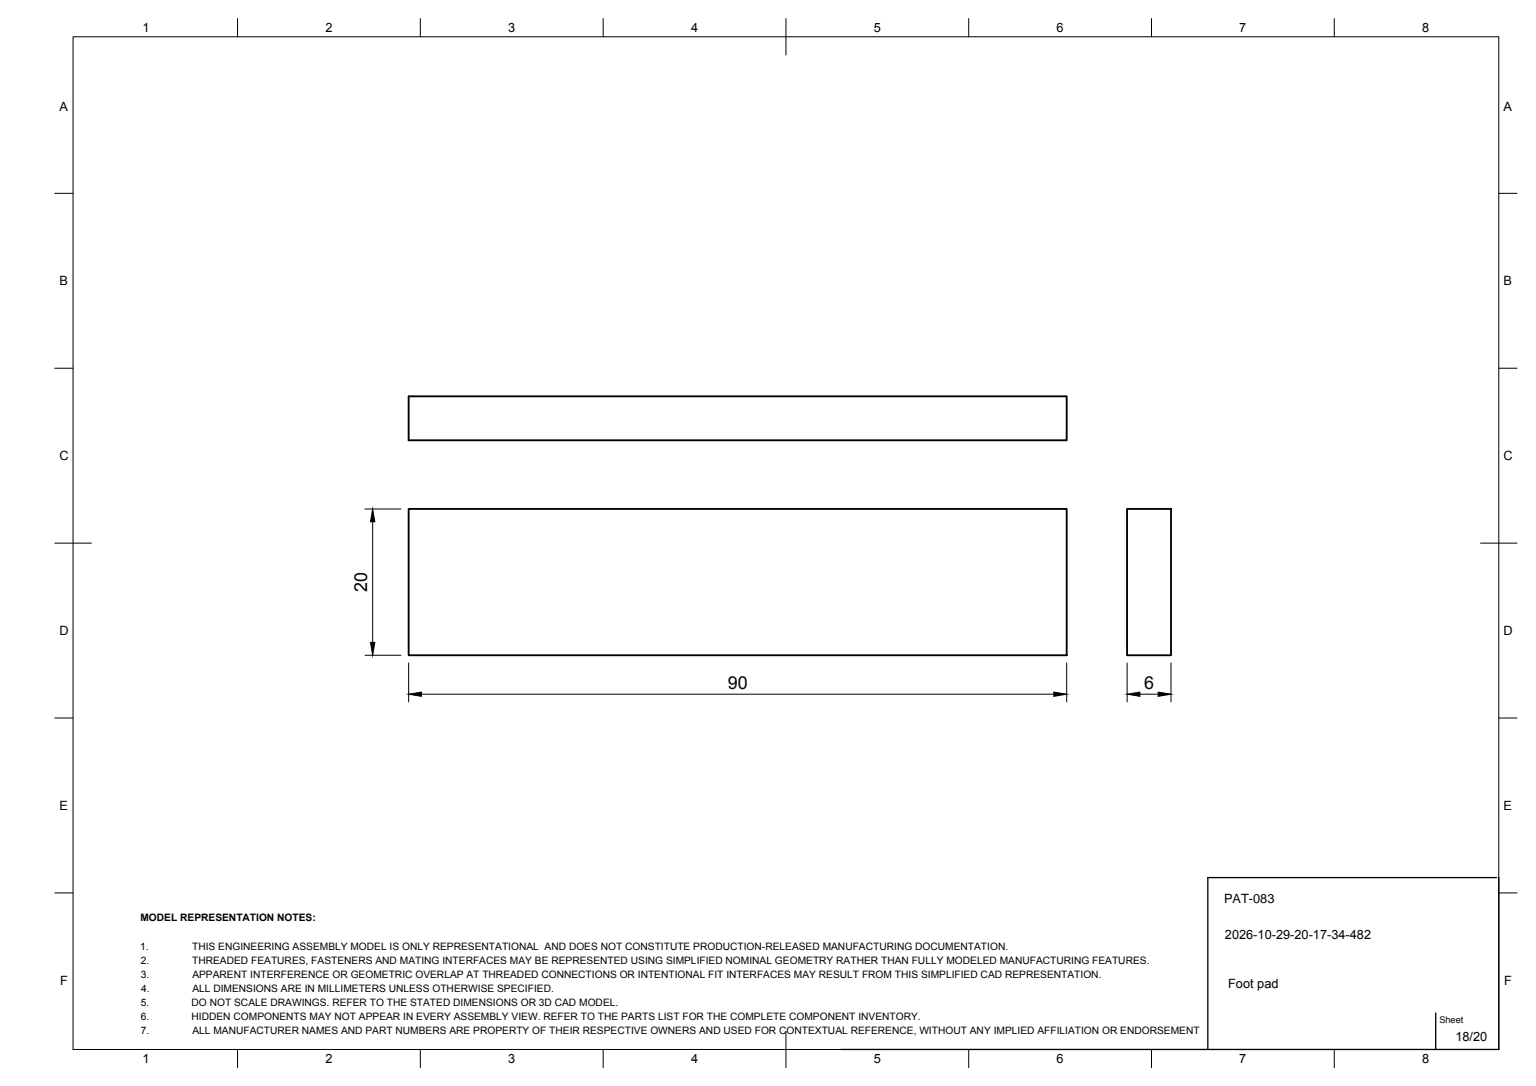
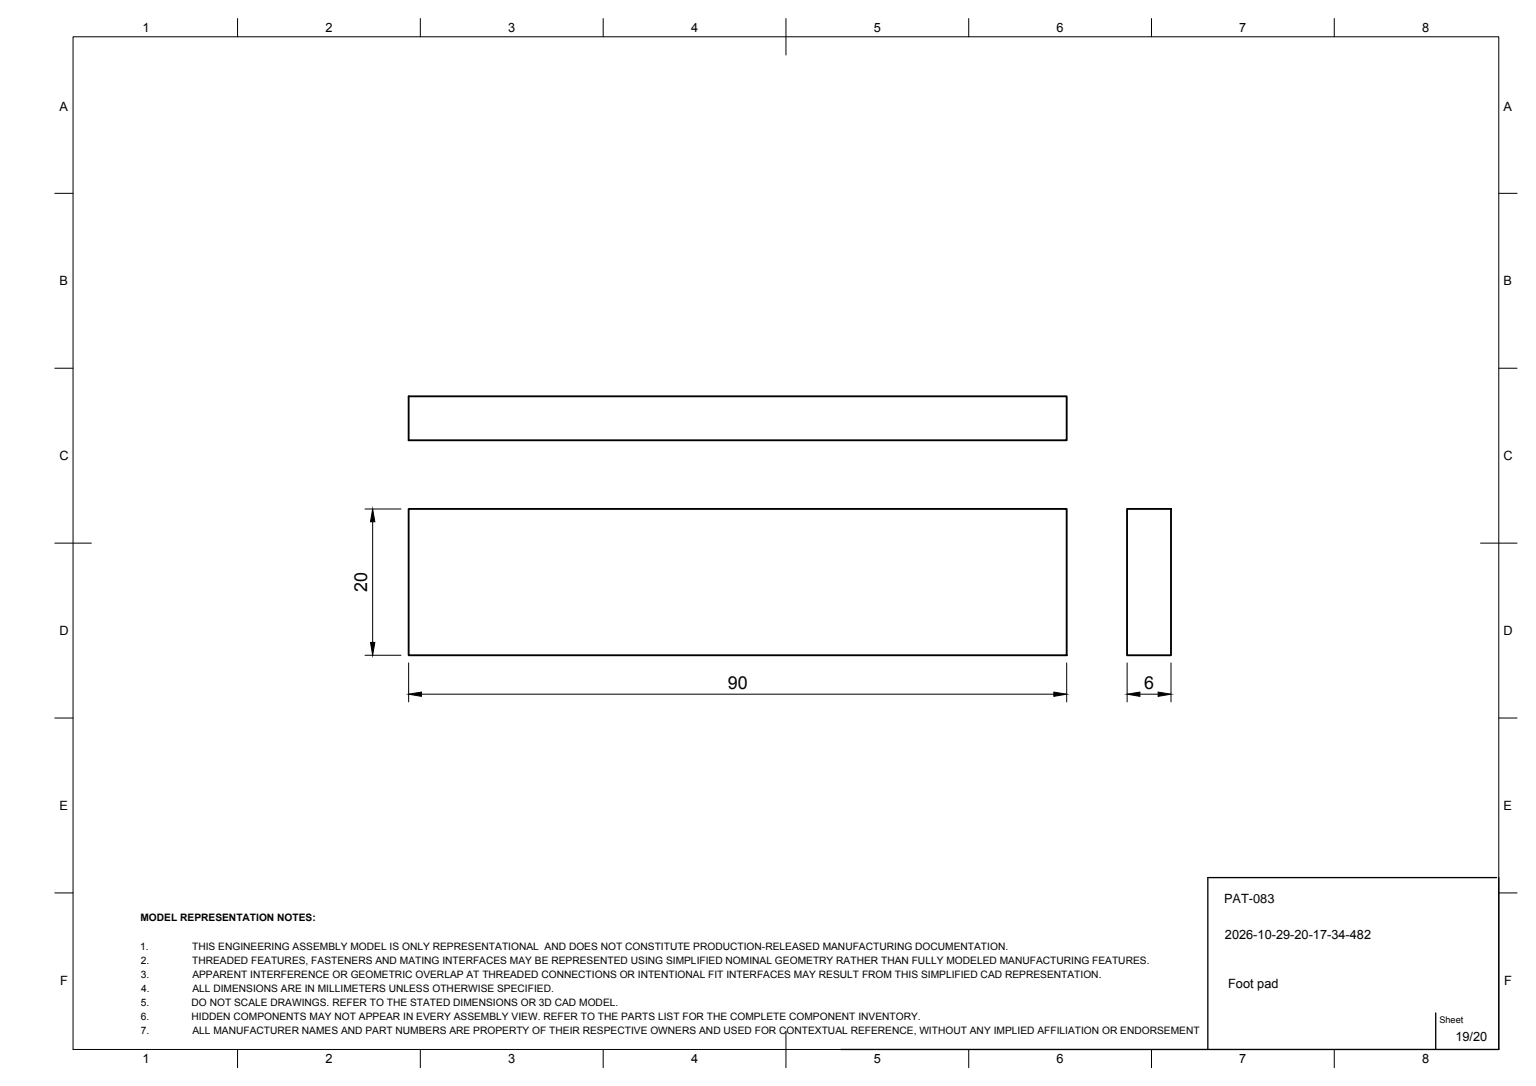
ISO-10303-21;
HEADER;
/* Generated by software containing ST-Developer
 * from STEP Tools, Inc. (www.steptools.com) 
 */

FILE_DESCRIPTION(
/* description */ ('PAT-083'),
/* implementation_level */ '2;1');

FILE_NAME(
/* name */ 'Foot pad.step',
/* time_stamp */ '2026-10-29T20:18:00-07:00',
/* author */ (''),
/* organization */ (''),
/* preprocessor_version */ 'ST-DEVELOPER v20.2',
/* originating_system */ 'Autodesk Translation Framework v15.17.0.0',
/* authorisation */ '');

FILE_SCHEMA (('AUTOMOTIVE_DESIGN { 1 0 10303 214 3 1 1 }'));
ENDSEC;

DATA;
#10=MECHANICAL_DESIGN_GEOMETRIC_PRESENTATION_REPRESENTATION('',(#245),#8428);
#197=SHAPE_REPRESENTATION_RELATIONSHIP('SRR','None',#8531,#221);
#221=ADVANCED_BREP_SHAPE_REPRESENTATION('',(#269),#8420);
#245=STYLED_ITEM('',(#8698),#269);
#269=MANIFOLD_SOLID_BREP('Body1',#3691);
#432=PLANE('',#4274);
#433=PLANE('',#4275);
#434=PLANE('',#4276);
#435=PLANE('',#4277);
#436=PLANE('',#4278);
#437=PLANE('',#4279);
#640=FACE_OUTER_BOUND('',#943,.T.);
#641=FACE_OUTER_BOUND('',#944,.T.);
#642=FACE_OUTER_BOUND('',#945,.T.);
#643=FACE_OUTER_BOUND('',#946,.T.);
#644=FACE_OUTER_BOUND('',#947,.T.);
#645=FACE_OUTER_BOUND('',#948,.T.);
#943=EDGE_LOOP('',(#3014,#3015,#3016,#3017));
#944=EDGE_LOOP('',(#3018,#3019,#3020,#3021));
#945=EDGE_LOOP('',(#3022,#3023,#3024,#3025));
#946=EDGE_LOOP('',(#3026,#3027,#3028,#3029));
#947=EDGE_LOOP('',(#3030,#3031,#3032,#3033));
#948=EDGE_LOOP('',(#3034,#3035,#3036,#3037));
#1159=LINE('',#7943,#1403);
#1160=LINE('',#7945,#1404);
#1161=LINE('',#7947,#1405);
#1162=LINE('',#7948,#1406);
#1163=LINE('',#7951,#1407);
#1164=LINE('',#7953,#1408);
#1165=LINE('',#7954,#1409);
#1166=LINE('',#7957,#1410);
#1167=LINE('',#7959,#1411);
#1168=LINE('',#7960,#1412);
#1169=LINE('',#7962,#1413);
#1170=LINE('',#7963,#1414);
#1403=VECTOR('',#5171,1.);
#1404=VECTOR('',#5172,1.);
#1405=VECTOR('',#5173,1.);
#1406=VECTOR('',#5174,1.);
#1407=VECTOR('',#5177,1.);
#1408=VECTOR('',#5178,1.);
#1409=VECTOR('',#5179,1.);
#1410=VECTOR('',#5182,1.);
#1411=VECTOR('',#5183,1.);
#1412=VECTOR('',#5184,1.);
#1413=VECTOR('',#5187,1.);
#1414=VECTOR('',#5188,1.);
#1893=VERTEX_POINT('',#7941);
#1894=VERTEX_POINT('',#7942);
#1895=VERTEX_POINT('',#7944);
#1896=VERTEX_POINT('',#7946);
#1897=VERTEX_POINT('',#7950);
#1898=VERTEX_POINT('',#7952);
#1899=VERTEX_POINT('',#7956);
#1900=VERTEX_POINT('',#7958);
#2283=EDGE_CURVE('',#1893,#1894,#1159,.T.);
#2284=EDGE_CURVE('',#1894,#1895,#1160,.T.);
#2285=EDGE_CURVE('',#1896,#1895,#1161,.T.);
#2286=EDGE_CURVE('',#1893,#1896,#1162,.T.);
#2287=EDGE_CURVE('',#1897,#1893,#1163,.T.);
#2288=EDGE_CURVE('',#1898,#1896,#1164,.T.);
#2289=EDGE_CURVE('',#1897,#1898,#1165,.T.);
#2290=EDGE_CURVE('',#1899,#1897,#1166,.T.);
#2291=EDGE_CURVE('',#1900,#1898,#1167,.T.);
#2292=EDGE_CURVE('',#1899,#1900,#1168,.T.);
#2293=EDGE_CURVE('',#1894,#1899,#1169,.T.);
#2294=EDGE_CURVE('',#1895,#1900,#1170,.T.);
#3014=ORIENTED_EDGE('',*,*,#2283,.T.);
#3015=ORIENTED_EDGE('',*,*,#2284,.T.);
#3016=ORIENTED_EDGE('',*,*,#2285,.F.);
#3017=ORIENTED_EDGE('',*,*,#2286,.F.);
#3018=ORIENTED_EDGE('',*,*,#2287,.T.);
#3019=ORIENTED_EDGE('',*,*,#2286,.T.);
#3020=ORIENTED_EDGE('',*,*,#2288,.F.);
#3021=ORIENTED_EDGE('',*,*,#2289,.F.);
#3022=ORIENTED_EDGE('',*,*,#2290,.T.);
#3023=ORIENTED_EDGE('',*,*,#2289,.T.);
#3024=ORIENTED_EDGE('',*,*,#2291,.F.);
#3025=ORIENTED_EDGE('',*,*,#2292,.F.);
#3026=ORIENTED_EDGE('',*,*,#2293,.T.);
#3027=ORIENTED_EDGE('',*,*,#2292,.T.);
#3028=ORIENTED_EDGE('',*,*,#2294,.F.);
#3029=ORIENTED_EDGE('',*,*,#2284,.F.);
#3030=ORIENTED_EDGE('',*,*,#2294,.T.);
#3031=ORIENTED_EDGE('',*,*,#2291,.T.);
#3032=ORIENTED_EDGE('',*,*,#2288,.T.);
#3033=ORIENTED_EDGE('',*,*,#2285,.T.);
#3034=ORIENTED_EDGE('',*,*,#2293,.F.);
#3035=ORIENTED_EDGE('',*,*,#2283,.F.);
#3036=ORIENTED_EDGE('',*,*,#2287,.F.);
#3037=ORIENTED_EDGE('',*,*,#2290,.F.);
#3587=ADVANCED_FACE('',(#640),#432,.T.);
#3588=ADVANCED_FACE('',(#641),#433,.T.);
#3589=ADVANCED_FACE('',(#642),#434,.T.);
#3590=ADVANCED_FACE('',(#643),#435,.T.);
#3591=ADVANCED_FACE('',(#644),#436,.T.);
#3592=ADVANCED_FACE('',(#645),#437,.F.);
#3691=CLOSED_SHELL('',(#3587,#3588,#3589,#3590,#3591,#3592));
#4273=AXIS2_PLACEMENT_3D('',#7939,#5167,#5168);
#4274=AXIS2_PLACEMENT_3D('',#7940,#5169,#5170);
#4275=AXIS2_PLACEMENT_3D('',#7949,#5175,#5176);
#4276=AXIS2_PLACEMENT_3D('',#7955,#5180,#5181);
#4277=AXIS2_PLACEMENT_3D('',#7961,#5185,#5186);
#4278=AXIS2_PLACEMENT_3D('',#7964,#5189,#5190);
#4279=AXIS2_PLACEMENT_3D('',#7965,#5191,#5192);
#5167=DIRECTION('axis',(0.,0.,1.));
#5168=DIRECTION('refdir',(1.,0.,0.));
#5169=DIRECTION('center_axis',(0.,1.,0.));
#5170=DIRECTION('ref_axis',(-1.,0.,0.));
#5171=DIRECTION('',(-1.,0.,0.));
#5172=DIRECTION('',(0.,0.,1.));
#5173=DIRECTION('',(-1.,0.,0.));
#5174=DIRECTION('',(0.,0.,1.));
#5175=DIRECTION('center_axis',(1.,0.,0.));
#5176=DIRECTION('ref_axis',(0.,1.,0.));
#5177=DIRECTION('',(0.,1.,0.));
#5178=DIRECTION('',(0.,1.,0.));
#5179=DIRECTION('',(0.,0.,1.));
#5180=DIRECTION('center_axis',(0.,-1.,0.));
#5181=DIRECTION('ref_axis',(1.,0.,0.));
#5182=DIRECTION('',(1.,0.,0.));
#5183=DIRECTION('',(1.,0.,0.));
#5184=DIRECTION('',(0.,0.,1.));
#5185=DIRECTION('center_axis',(-1.,0.,0.));
#5186=DIRECTION('ref_axis',(0.,-1.,0.));
#5187=DIRECTION('',(0.,-1.,0.));
#5188=DIRECTION('',(0.,-1.,0.));
#5189=DIRECTION('center_axis',(0.,0.,1.));
#5190=DIRECTION('ref_axis',(1.,0.,0.));
#5191=DIRECTION('center_axis',(0.,0.,1.));
#5192=DIRECTION('ref_axis',(1.,0.,0.));
#7939=CARTESIAN_POINT('',(0.,0.,0.));
#7940=CARTESIAN_POINT('Origin',(-4.,4.5,-0.6));
#7941=CARTESIAN_POINT('',(-4.,4.5,-0.6));
#7942=CARTESIAN_POINT('',(-6.,4.5,-0.6));
#7943=CARTESIAN_POINT('',(-4.,4.5,-0.6));
#7944=CARTESIAN_POINT('',(-6.,4.5,0.));
#7945=CARTESIAN_POINT('',(-6.,4.5,-0.6));
#7946=CARTESIAN_POINT('',(-4.,4.5,0.));
#7947=CARTESIAN_POINT('',(-4.,4.5,0.));
#7948=CARTESIAN_POINT('',(-4.,4.5,-0.6));
#7949=CARTESIAN_POINT('Origin',(-4.,-4.5,-0.6));
#7950=CARTESIAN_POINT('',(-4.,-4.5,-0.6));
#7951=CARTESIAN_POINT('',(-4.,-4.5,-0.6));
#7952=CARTESIAN_POINT('',(-4.,-4.5,0.));
#7953=CARTESIAN_POINT('',(-4.,-4.5,0.));
#7954=CARTESIAN_POINT('',(-4.,-4.5,-0.6));
#7955=CARTESIAN_POINT('Origin',(-6.,-4.5,-0.6));
#7956=CARTESIAN_POINT('',(-6.,-4.5,-0.6));
#7957=CARTESIAN_POINT('',(-6.,-4.5,-0.6));
#7958=CARTESIAN_POINT('',(-6.,-4.5,0.));
#7959=CARTESIAN_POINT('',(-6.,-4.5,0.));
#7960=CARTESIAN_POINT('',(-6.,-4.5,-0.6));
#7961=CARTESIAN_POINT('Origin',(-6.,4.5,-0.6));
#7962=CARTESIAN_POINT('',(-6.,4.5,-0.6));
#7963=CARTESIAN_POINT('',(-6.,4.5,0.));
#7964=CARTESIAN_POINT('Origin',(-5.,0.,0.));
#7965=CARTESIAN_POINT('Origin',(-5.,0.,-0.6));
#8394=UNCERTAINTY_MEASURE_WITH_UNIT(LENGTH_MEASURE(0.001),#8429,
'DISTANCE_ACCURACY_VALUE',
'Maximum model space distance between geometric entities at asserted c
onnectivities');
#8402=UNCERTAINTY_MEASURE_WITH_UNIT(LENGTH_MEASURE(0.001),#8429,
'DISTANCE_ACCURACY_VALUE',
'Maximum model space distance between geometric entities at asserted c
onnectivities');
#8420=(
GEOMETRIC_REPRESENTATION_CONTEXT(3)
GLOBAL_UNCERTAINTY_ASSIGNED_CONTEXT((#8394))
GLOBAL_UNIT_ASSIGNED_CONTEXT((#8429,#8431,#8432))
REPRESENTATION_CONTEXT('','3D')
);
#8428=(
GEOMETRIC_REPRESENTATION_CONTEXT(3)
GLOBAL_UNCERTAINTY_ASSIGNED_CONTEXT((#8402))
GLOBAL_UNIT_ASSIGNED_CONTEXT((#8429,#8431,#8432))
REPRESENTATION_CONTEXT('','3D')
);
#8429=(
LENGTH_UNIT()
NAMED_UNIT(*)
SI_UNIT(.CENTI.,.METRE.)
);
#8431=(
NAMED_UNIT(*)
PLANE_ANGLE_UNIT()
SI_UNIT($,.RADIAN.)
);
#8432=(
NAMED_UNIT(*)
SI_UNIT($,.STERADIAN.)
SOLID_ANGLE_UNIT()
);
#8450=SHAPE_DEFINITION_REPRESENTATION(#8475,#8531);
#8475=PRODUCT_DEFINITION_SHAPE('',$,#8557);
#8531=SHAPE_REPRESENTATION('',(#4273),#8420);
#8539=PRODUCT_DEFINITION_CONTEXT('part definition',#8616,'design');
#8557=PRODUCT_DEFINITION('Foot pad','Foot pad',#8582,#8539);
#8582=PRODUCT_DEFINITION_FORMATION('',$,#8635);
#8616=APPLICATION_CONTEXT(
'Core Data for Automotive Mechanical Design Process');
#8617=PRODUCT_CONTEXT('part definition',#8616,'mechanical');
#8635=PRODUCT('Foot pad','Foot pad','Foot pad',(#8617));
#8692=COLOUR_RGB('Sky Blue',0.24,0.69,0.87);
#8693=FILL_AREA_STYLE_COLOUR('',#8692);
#8694=FILL_AREA_STYLE('',(#8693));
#8695=SURFACE_STYLE_FILL_AREA(#8694);
#8696=SURFACE_SIDE_STYLE('',(#8695));
#8697=SURFACE_STYLE_USAGE(.BOTH.,#8696);
#8698=PRESENTATION_STYLE_ASSIGNMENT((#8697));
ENDSEC;
END-ISO-10303-21;
